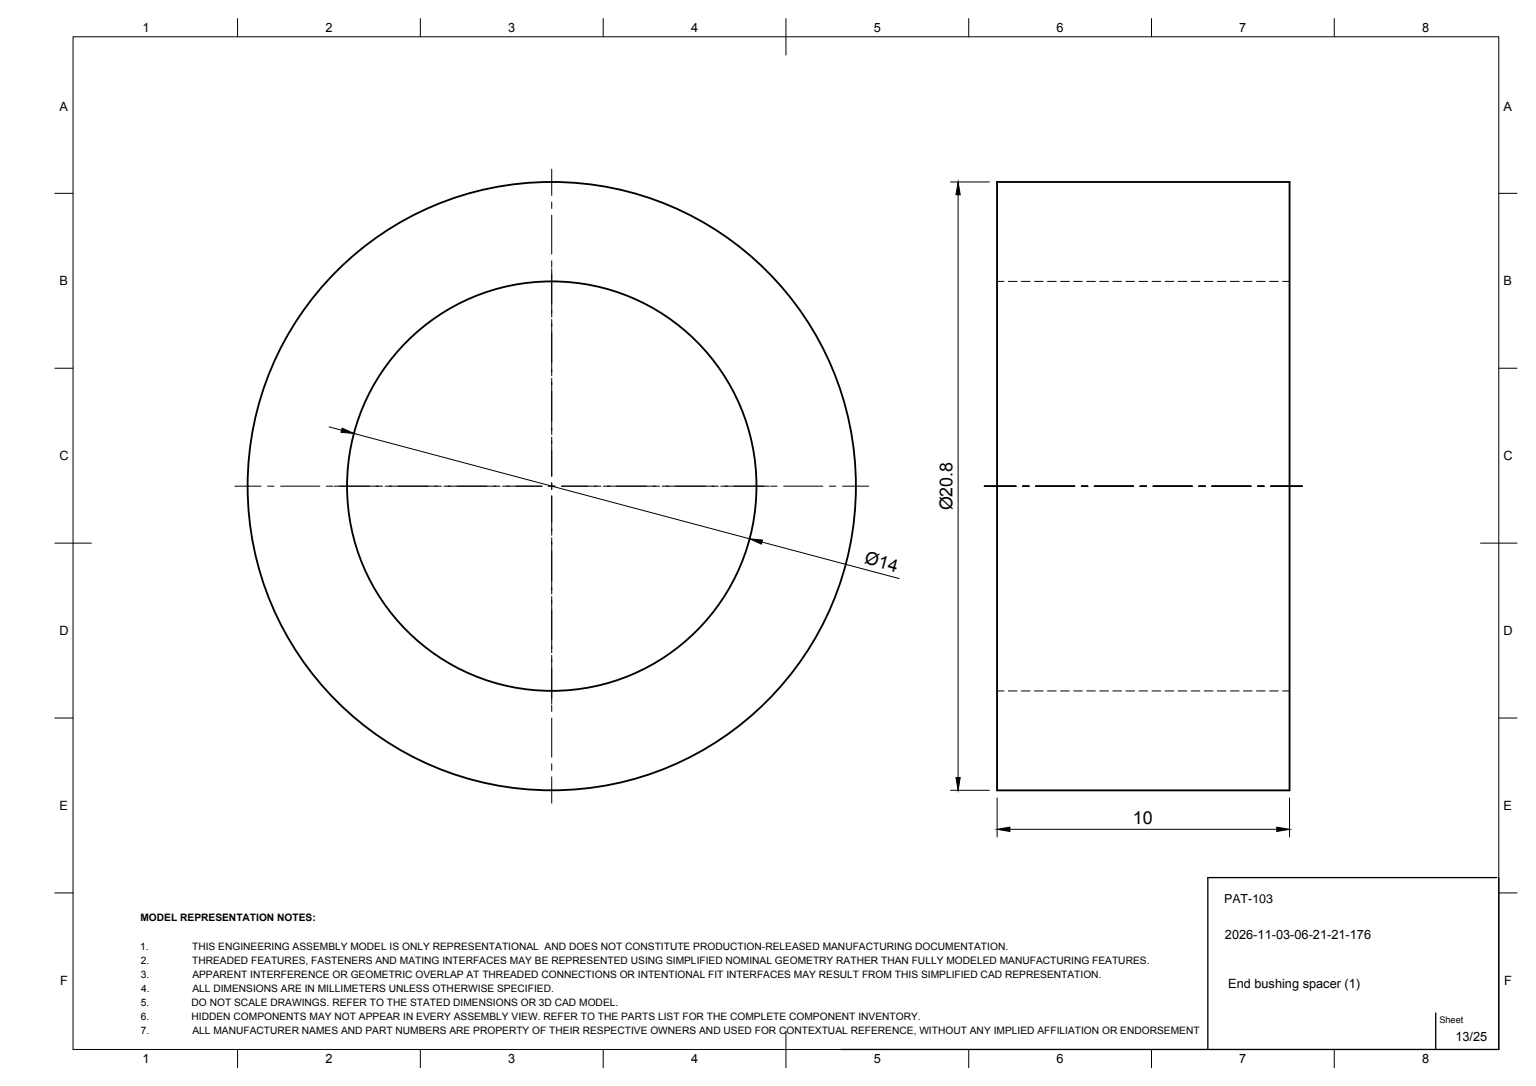
ISO-10303-21;
HEADER;
/* Generated by software containing ST-Developer
 * from STEP Tools, Inc. (www.steptools.com) 
 */

FILE_DESCRIPTION(
/* description */ ('Telescoping shaft support with lock collar'),
/* implementation_level */ '2;1');

FILE_NAME(
/* name */ 'End bushing spacer (1).step',
/* time_stamp */ '2026-10-27T10:48:51-07:00',
/* author */ (''),
/* organization */ (''),
/* preprocessor_version */ 'ST-DEVELOPER v20.2',
/* originating_system */ 'Autodesk Translation Framework v15.17.0.0',
/* authorisation */ '');

FILE_SCHEMA (('AUTOMOTIVE_DESIGN { 1 0 10303 214 3 1 1 }'));
ENDSEC;

DATA;
#10=MECHANICAL_DESIGN_GEOMETRIC_PRESENTATION_REPRESENTATION('',(#249),#7349);
#209=SHAPE_REPRESENTATION_RELATIONSHIP('SRR','None',#7451,#229);
#229=ADVANCED_BREP_SHAPE_REPRESENTATION('',(#269),#7335);
#249=STYLED_ITEM('',(#7641),#269);
#269=MANIFOLD_SOLID_BREP('Body1',#3972);
#317=FACE_BOUND('',#860,.T.);
#318=FACE_BOUND('',#862,.T.);
#419=PLANE('',#4422);
#420=PLANE('',#4423);
#593=FACE_OUTER_BOUND('',#857,.T.);
#594=FACE_OUTER_BOUND('',#858,.T.);
#595=FACE_OUTER_BOUND('',#859,.T.);
#596=FACE_OUTER_BOUND('',#861,.T.);
#857=EDGE_LOOP('',(#3110,#3111,#3112,#3113));
#858=EDGE_LOOP('',(#3114,#3115,#3116,#3117));
#859=EDGE_LOOP('',(#3118));
#860=EDGE_LOOP('',(#3119));
#861=EDGE_LOOP('',(#3120));
#862=EDGE_LOOP('',(#3121));
#1161=LINE('',#6490,#1441);
#1162=LINE('',#6496,#1442);
#1441=VECTOR('',#5263,0.7);
#1442=VECTOR('',#5270,1.04);
#1687=CIRCLE('',#4417,0.7);
#1688=CIRCLE('',#4418,0.7);
#1689=CIRCLE('',#4420,1.04);
#1690=CIRCLE('',#4421,1.04);
#1954=VERTEX_POINT('',#6487);
#1955=VERTEX_POINT('',#6489);
#1956=VERTEX_POINT('',#6493);
#1957=VERTEX_POINT('',#6495);
#2367=EDGE_CURVE('',#1954,#1954,#1687,.T.);
#2368=EDGE_CURVE('',#1954,#1955,#1161,.T.);
#2369=EDGE_CURVE('',#1955,#1955,#1688,.T.);
#2370=EDGE_CURVE('',#1956,#1956,#1689,.T.);
#2371=EDGE_CURVE('',#1956,#1957,#1162,.T.);
#2372=EDGE_CURVE('',#1957,#1957,#1690,.T.);
#3110=ORIENTED_EDGE('',*,*,#2367,.F.);
#3111=ORIENTED_EDGE('',*,*,#2368,.T.);
#3112=ORIENTED_EDGE('',*,*,#2369,.T.);
#3113=ORIENTED_EDGE('',*,*,#2368,.F.);
#3114=ORIENTED_EDGE('',*,*,#2370,.F.);
#3115=ORIENTED_EDGE('',*,*,#2371,.T.);
#3116=ORIENTED_EDGE('',*,*,#2372,.T.);
#3117=ORIENTED_EDGE('',*,*,#2371,.F.);
#3118=ORIENTED_EDGE('',*,*,#2370,.T.);
#3119=ORIENTED_EDGE('',*,*,#2367,.T.);
#3120=ORIENTED_EDGE('',*,*,#2372,.F.);
#3121=ORIENTED_EDGE('',*,*,#2369,.F.);
#3698=CYLINDRICAL_SURFACE('',#4416,0.7);
#3699=CYLINDRICAL_SURFACE('',#4419,1.04);
#3836=ADVANCED_FACE('',(#593),#3698,.F.);
#3837=ADVANCED_FACE('',(#594),#3699,.T.);
#3838=ADVANCED_FACE('',(#595,#317),#419,.T.);
#3839=ADVANCED_FACE('',(#596,#318),#420,.F.);
#3972=CLOSED_SHELL('',(#3836,#3837,#3838,#3839));
#4415=AXIS2_PLACEMENT_3D('',#6485,#5257,#5258);
#4416=AXIS2_PLACEMENT_3D('',#6486,#5259,#5260);
#4417=AXIS2_PLACEMENT_3D('',#6488,#5261,#5262);
#4418=AXIS2_PLACEMENT_3D('',#6491,#5264,#5265);
#4419=AXIS2_PLACEMENT_3D('',#6492,#5266,#5267);
#4420=AXIS2_PLACEMENT_3D('',#6494,#5268,#5269);
#4421=AXIS2_PLACEMENT_3D('',#6497,#5271,#5272);
#4422=AXIS2_PLACEMENT_3D('',#6498,#5273,#5274);
#4423=AXIS2_PLACEMENT_3D('',#6499,#5275,#5276);
#5257=DIRECTION('axis',(0.,0.,1.));
#5258=DIRECTION('refdir',(1.,0.,0.));
#5259=DIRECTION('center_axis',(1.,0.,0.));
#5260=DIRECTION('ref_axis',(0.,0.,-1.));
#5261=DIRECTION('center_axis',(-1.,0.,0.));
#5262=DIRECTION('ref_axis',(0.,0.,-1.));
#5263=DIRECTION('',(-1.,0.,0.));
#5264=DIRECTION('center_axis',(-1.,0.,0.));
#5265=DIRECTION('ref_axis',(0.,0.,-1.));
#5266=DIRECTION('center_axis',(1.,0.,0.));
#5267=DIRECTION('ref_axis',(0.,0.,-1.));
#5268=DIRECTION('center_axis',(1.,0.,0.));
#5269=DIRECTION('ref_axis',(0.,0.,-1.));
#5270=DIRECTION('',(-1.,0.,0.));
#5271=DIRECTION('center_axis',(1.,0.,0.));
#5272=DIRECTION('ref_axis',(0.,0.,-1.));
#5273=DIRECTION('center_axis',(1.,0.,0.));
#5274=DIRECTION('ref_axis',(0.,0.,-1.));
#5275=DIRECTION('center_axis',(1.,0.,0.));
#5276=DIRECTION('ref_axis',(0.,0.,-1.));
#6485=CARTESIAN_POINT('',(0.,0.,0.));
#6486=CARTESIAN_POINT('Origin',(9.,0.,3.5));
#6487=CARTESIAN_POINT('',(10.,-8.57252759403147E-17,4.2));
#6488=CARTESIAN_POINT('Origin',(10.,0.,3.5));
#6489=CARTESIAN_POINT('',(9.,-8.57252759403147E-17,4.2));
#6490=CARTESIAN_POINT('',(9.,-8.57252759403147E-17,4.2));
#6491=CARTESIAN_POINT('Origin',(9.,0.,3.5));
#6492=CARTESIAN_POINT('Origin',(9.,0.,3.5));
#6493=CARTESIAN_POINT('',(10.,-1.27363267111325E-16,4.54));
#6494=CARTESIAN_POINT('Origin',(10.,0.,3.5));
#6495=CARTESIAN_POINT('',(9.,-1.27363267111325E-16,4.54));
#6496=CARTESIAN_POINT('',(9.,-1.27363267111325E-16,4.54));
#6497=CARTESIAN_POINT('Origin',(9.,0.,3.5));
#6498=CARTESIAN_POINT('Origin',(10.,0.,3.5));
#6499=CARTESIAN_POINT('Origin',(9.,0.,3.5));
#7310=UNCERTAINTY_MEASURE_WITH_UNIT(LENGTH_MEASURE(0.001),#7350,
'DISTANCE_ACCURACY_VALUE',
'Maximum model space distance between geometric entities at asserted c
onnectivities');
#7324=UNCERTAINTY_MEASURE_WITH_UNIT(LENGTH_MEASURE(0.001),#7350,
'DISTANCE_ACCURACY_VALUE',
'Maximum model space distance between geometric entities at asserted c
onnectivities');
#7335=(
GEOMETRIC_REPRESENTATION_CONTEXT(3)
GLOBAL_UNCERTAINTY_ASSIGNED_CONTEXT((#7310))
GLOBAL_UNIT_ASSIGNED_CONTEXT((#7350,#7352,#7353))
REPRESENTATION_CONTEXT('','3D')
);
#7349=(
GEOMETRIC_REPRESENTATION_CONTEXT(3)
GLOBAL_UNCERTAINTY_ASSIGNED_CONTEXT((#7324))
GLOBAL_UNIT_ASSIGNED_CONTEXT((#7350,#7352,#7353))
REPRESENTATION_CONTEXT('','3D')
);
#7350=(
LENGTH_UNIT()
NAMED_UNIT(*)
SI_UNIT(.CENTI.,.METRE.)
);
#7352=(
NAMED_UNIT(*)
PLANE_ANGLE_UNIT()
SI_UNIT($,.RADIAN.)
);
#7353=(
NAMED_UNIT(*)
SI_UNIT($,.STERADIAN.)
SOLID_ANGLE_UNIT()
);
#7364=SHAPE_DEFINITION_REPRESENTATION(#7388,#7451);
#7388=PRODUCT_DEFINITION_SHAPE('',$,#7476);
#7451=SHAPE_REPRESENTATION('',(#4415),#7335);
#7465=PRODUCT_DEFINITION_CONTEXT('part definition',#7539,'design');
#7476=PRODUCT_DEFINITION('End bushing spacer (1)',
'End bushing spacer (1)',#7500,#7465);
#7500=PRODUCT_DEFINITION_FORMATION('',$,#7551);
#7539=APPLICATION_CONTEXT(
'Core Data for Automotive Mechanical Design Process');
#7540=PRODUCT_CONTEXT('part definition',#7539,'mechanical');
#7551=PRODUCT('End bushing spacer (1)','End bushing spacer (1)',
'End bushing spacer (1)',(#7540));
#7635=COLOUR_RGB('Off White',0.89,0.88,0.83);
#7636=FILL_AREA_STYLE_COLOUR('',#7635);
#7637=FILL_AREA_STYLE('',(#7636));
#7638=SURFACE_STYLE_FILL_AREA(#7637);
#7639=SURFACE_SIDE_STYLE('',(#7638));
#7640=SURFACE_STYLE_USAGE(.BOTH.,#7639);
#7641=PRESENTATION_STYLE_ASSIGNMENT((#7640));
ENDSEC;
END-ISO-10303-21;
